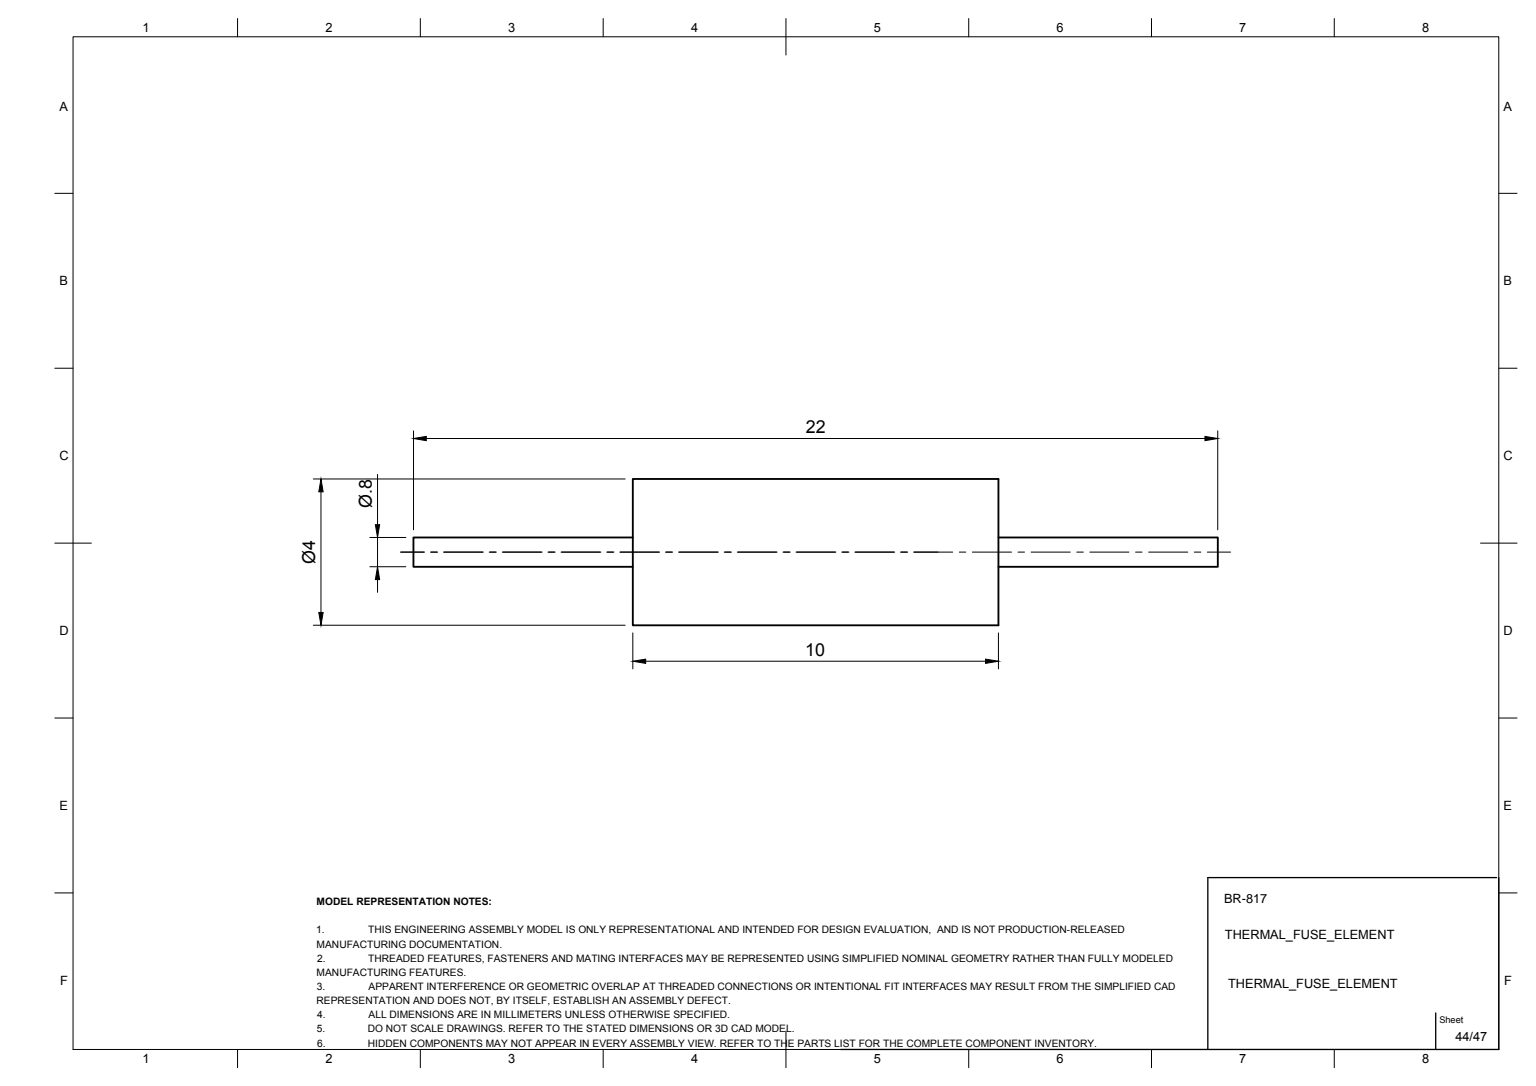
ISO-10303-21;
HEADER;
FILE_DESCRIPTION((''),'2;1');
FILE_NAME('THERMAL_FUSE_ELEMENT.step','2026-10-01T22:07:29-07:00',(''),(''),'','','');
FILE_SCHEMA (('AUTOMOTIVE_DESIGN { 1 0 10303 214 3 1 1 }'));
ENDSEC;
DATA;
#10=MECHANICAL_DESIGN_GEOMETRIC_PRESENTATION_REPRESENTATION('',(#579,#580,#581),#15484);
#504=SHAPE_REPRESENTATION_RELATIONSHIP('SRR','None',#15655,#539) ;
#539=ADVANCED_BREP_SHAPE_REPRESENTATION('',(#620,#621,#622),#15479) ;
#579=STYLED_ITEM('',(#15835),#620) ;
#580=STYLED_ITEM('',(#15842),#621) ;
#581=STYLED_ITEM('',(#15842),#622) ;
#620=MANIFOLD_SOLID_BREP('FUSE_BODY',#8290) ;
#621=MANIFOLD_SOLID_BREP('FUSE_LEADS',#8291) ;
#622=MANIFOLD_SOLID_BREP('FUSE_LEADS',#8292) ;
#802=CYLINDRICAL_SURFACE('',#9864,0.2) ;
#803=CYLINDRICAL_SURFACE('',#9869,0.04) ;
#804=CYLINDRICAL_SURFACE('',#9874,0.04) ;
#1349=CIRCLE('',#9865,0.2) ;
#1350=CIRCLE('',#9866,0.2) ;
#1351=CIRCLE('',#9870,0.04) ;
#1352=CIRCLE('',#9871,0.04) ;
#1353=CIRCLE('',#9875,0.04) ;
#1354=CIRCLE('',#9876,0.04) ;
#1843=FACE_OUTER_BOUND('',#2416,.T.) ;
#1844=FACE_OUTER_BOUND('',#2417,.T.) ;
#1845=FACE_OUTER_BOUND('',#2418,.T.) ;
#1846=FACE_OUTER_BOUND('',#2419,.T.) ;
#1847=FACE_OUTER_BOUND('',#2420,.T.) ;
#1848=FACE_OUTER_BOUND('',#2421,.T.) ;
#1849=FACE_OUTER_BOUND('',#2422,.T.) ;
#1850=FACE_OUTER_BOUND('',#2423,.T.) ;
#1851=FACE_OUTER_BOUND('',#2424,.T.) ;
#2416=EDGE_LOOP('',(#7489,#7490,#7491,#7492)) ;
#2417=EDGE_LOOP('',(#7493)) ;
#2418=EDGE_LOOP('',(#7494)) ;
#2419=EDGE_LOOP('',(#7495,#7496,#7497,#7498)) ;
#2420=EDGE_LOOP('',(#7499)) ;
#2421=EDGE_LOOP('',(#7500)) ;
#2422=EDGE_LOOP('',(#7501,#7502,#7503,#7504)) ;
#2423=EDGE_LOOP('',(#7505)) ;
#2424=EDGE_LOOP('',(#7506)) ;
#2906=LINE('',#15318,#3380) ;
#2907=LINE('',#15326,#3381) ;
#2908=LINE('',#15334,#3382) ;
#3380=VECTOR('',#12759,0.2) ;
#3381=VECTOR('',#12770,0.04) ;
#3382=VECTOR('',#12781,0.04) ;
#4125=VERTEX_POINT('',#15315) ;
#4126=VERTEX_POINT('',#15317) ;
#4127=VERTEX_POINT('',#15323) ;
#4128=VERTEX_POINT('',#15325) ;
#4129=VERTEX_POINT('',#15331) ;
#4130=VERTEX_POINT('',#15333) ;
#5249=EDGE_CURVE('',#4125,#4125,#1349,.T.) ;
#5250=EDGE_CURVE('',#4125,#4126,#2906,.T.) ;
#5251=EDGE_CURVE('',#4126,#4126,#1350,.T.) ;
#5252=EDGE_CURVE('',#4127,#4127,#1351,.T.) ;
#5253=EDGE_CURVE('',#4127,#4128,#2907,.T.) ;
#5254=EDGE_CURVE('',#4128,#4128,#1352,.T.) ;
#5255=EDGE_CURVE('',#4129,#4129,#1353,.T.) ;
#5256=EDGE_CURVE('',#4129,#4130,#2908,.T.) ;
#5257=EDGE_CURVE('',#4130,#4130,#1354,.T.) ;
#7489=ORIENTED_EDGE('',*,*,#5249,.F.) ;
#7490=ORIENTED_EDGE('',*,*,#5250,.T.) ;
#7491=ORIENTED_EDGE('',*,*,#5251,.F.) ;
#7492=ORIENTED_EDGE('',*,*,#5250,.F.) ;
#7493=ORIENTED_EDGE('',*,*,#5251,.T.) ;
#7494=ORIENTED_EDGE('',*,*,#5249,.T.) ;
#7495=ORIENTED_EDGE('',*,*,#5252,.F.) ;
#7496=ORIENTED_EDGE('',*,*,#5253,.T.) ;
#7497=ORIENTED_EDGE('',*,*,#5254,.F.) ;
#7498=ORIENTED_EDGE('',*,*,#5253,.F.) ;
#7499=ORIENTED_EDGE('',*,*,#5254,.T.) ;
#7500=ORIENTED_EDGE('',*,*,#5252,.T.) ;
#7501=ORIENTED_EDGE('',*,*,#5255,.F.) ;
#7502=ORIENTED_EDGE('',*,*,#5256,.T.) ;
#7503=ORIENTED_EDGE('',*,*,#5257,.F.) ;
#7504=ORIENTED_EDGE('',*,*,#5256,.F.) ;
#7505=ORIENTED_EDGE('',*,*,#5257,.T.) ;
#7506=ORIENTED_EDGE('',*,*,#5255,.T.) ;
#7738=PLANE('',#9867) ;
#7739=PLANE('',#9868) ;
#7740=PLANE('',#9872) ;
#7741=PLANE('',#9873) ;
#7742=PLANE('',#9877) ;
#7743=PLANE('',#9878) ;
#8230=ADVANCED_FACE('',(#1843),#802,.T.) ;
#8231=ADVANCED_FACE('',(#1844),#7738,.T.) ;
#8232=ADVANCED_FACE('',(#1845),#7739,.T.) ;
#8233=ADVANCED_FACE('',(#1846),#803,.T.) ;
#8234=ADVANCED_FACE('',(#1847),#7740,.T.) ;
#8235=ADVANCED_FACE('',(#1848),#7741,.T.) ;
#8236=ADVANCED_FACE('',(#1849),#804,.T.) ;
#8237=ADVANCED_FACE('',(#1850),#7742,.T.) ;
#8238=ADVANCED_FACE('',(#1851),#7743,.T.) ;
#8290=CLOSED_SHELL('',(#8230,#8231,#8232)) ;
#8291=CLOSED_SHELL('',(#8233,#8234,#8235)) ;
#8292=CLOSED_SHELL('',(#8236,#8237,#8238)) ;
#9863=AXIS2_PLACEMENT_3D('',#15313,#12753,#12754) ;
#9864=AXIS2_PLACEMENT_3D('',#15314,#12755,#12756) ;
#9865=AXIS2_PLACEMENT_3D('',#15316,#12757,#12758) ;
#9866=AXIS2_PLACEMENT_3D('',#15319,#12760,#12761) ;
#9867=AXIS2_PLACEMENT_3D('',#15320,#12762,#12763) ;
#9868=AXIS2_PLACEMENT_3D('',#15321,#12764,#12765) ;
#9869=AXIS2_PLACEMENT_3D('',#15322,#12766,#12767) ;
#9870=AXIS2_PLACEMENT_3D('',#15324,#12768,#12769) ;
#9871=AXIS2_PLACEMENT_3D('',#15327,#12771,#12772) ;
#9872=AXIS2_PLACEMENT_3D('',#15328,#12773,#12774) ;
#9873=AXIS2_PLACEMENT_3D('',#15329,#12775,#12776) ;
#9874=AXIS2_PLACEMENT_3D('',#15330,#12777,#12778) ;
#9875=AXIS2_PLACEMENT_3D('',#15332,#12779,#12780) ;
#9876=AXIS2_PLACEMENT_3D('',#15335,#12782,#12783) ;
#9877=AXIS2_PLACEMENT_3D('',#15336,#12784,#12785) ;
#9878=AXIS2_PLACEMENT_3D('',#15337,#12786,#12787) ;
#12753=DIRECTION('axis',(0.,0.,1.)) ;
#12754=DIRECTION('refdir',(1.,0.,0.)) ;
#12755=DIRECTION('center_axis',(1.,0.,0.)) ;
#12756=DIRECTION('ref_axis',(0.,0.,-1.)) ;
#12757=DIRECTION('center_axis',(1.,0.,0.)) ;
#12758=DIRECTION('ref_axis',(0.,0.,-1.)) ;
#12759=DIRECTION('',(-1.,0.,0.)) ;
#12760=DIRECTION('center_axis',(-1.,0.,0.)) ;
#12761=DIRECTION('ref_axis',(0.,0.,-1.)) ;
#12762=DIRECTION('center_axis',(-1.,0.,0.)) ;
#12763=DIRECTION('ref_axis',(0.,0.,1.)) ;
#12764=DIRECTION('center_axis',(1.,0.,0.)) ;
#12765=DIRECTION('ref_axis',(0.,0.,-1.)) ;
#12766=DIRECTION('center_axis',(1.,0.,0.)) ;
#12767=DIRECTION('ref_axis',(0.,0.,-1.)) ;
#12768=DIRECTION('center_axis',(1.,0.,0.)) ;
#12769=DIRECTION('ref_axis',(0.,0.,-1.)) ;
#12770=DIRECTION('',(-1.,0.,0.)) ;
#12771=DIRECTION('center_axis',(-1.,0.,0.)) ;
#12772=DIRECTION('ref_axis',(0.,0.,-1.)) ;
#12773=DIRECTION('center_axis',(-1.,0.,0.)) ;
#12774=DIRECTION('ref_axis',(0.,0.,1.)) ;
#12775=DIRECTION('center_axis',(1.,0.,0.)) ;
#12776=DIRECTION('ref_axis',(0.,0.,-1.)) ;
#12777=DIRECTION('center_axis',(1.,0.,0.)) ;
#12778=DIRECTION('ref_axis',(0.,0.,-1.)) ;
#12779=DIRECTION('center_axis',(1.,0.,0.)) ;
#12780=DIRECTION('ref_axis',(0.,0.,-1.)) ;
#12781=DIRECTION('',(-1.,0.,0.)) ;
#12782=DIRECTION('center_axis',(-1.,0.,0.)) ;
#12783=DIRECTION('ref_axis',(0.,0.,-1.)) ;
#12784=DIRECTION('center_axis',(-1.,0.,0.)) ;
#12785=DIRECTION('ref_axis',(0.,0.,1.)) ;
#12786=DIRECTION('center_axis',(1.,0.,0.)) ;
#12787=DIRECTION('ref_axis',(0.,0.,-1.)) ;
#15313=CARTESIAN_POINT('',(0.,0.,0.)) ;
#15314=CARTESIAN_POINT('Origin',(1.6,-1.8,0.6)) ;
#15315=CARTESIAN_POINT('',(2.1,-1.8,0.8)) ;
#15316=CARTESIAN_POINT('Origin',(2.1,-1.8,0.6)) ;
#15317=CARTESIAN_POINT('',(1.1,-1.8,0.8)) ;
#15318=CARTESIAN_POINT('',(1.6,-1.8,0.8)) ;
#15319=CARTESIAN_POINT('Origin',(1.1,-1.8,0.6)) ;
#15320=CARTESIAN_POINT('Origin',(1.1,-1.8,0.6)) ;
#15321=CARTESIAN_POINT('Origin',(2.1,-1.8,0.6)) ;
#15322=CARTESIAN_POINT('Origin',(0.8,-1.8,0.6)) ;
#15323=CARTESIAN_POINT('',(1.1,-1.8,0.64)) ;
#15324=CARTESIAN_POINT('Origin',(1.1,-1.8,0.6)) ;
#15325=CARTESIAN_POINT('',(0.5,-1.8,0.64)) ;
#15326=CARTESIAN_POINT('',(0.8,-1.8,0.64)) ;
#15327=CARTESIAN_POINT('Origin',(0.5,-1.8,0.6)) ;
#15328=CARTESIAN_POINT('Origin',(0.5,-1.8,0.6)) ;
#15329=CARTESIAN_POINT('Origin',(1.1,-1.8,0.6)) ;
#15330=CARTESIAN_POINT('Origin',(2.4,-1.8,0.6)) ;
#15331=CARTESIAN_POINT('',(2.7,-1.8,0.64)) ;
#15332=CARTESIAN_POINT('Origin',(2.7,-1.8,0.6)) ;
#15333=CARTESIAN_POINT('',(2.1,-1.8,0.64)) ;
#15334=CARTESIAN_POINT('',(2.4,-1.8,0.64)) ;
#15335=CARTESIAN_POINT('Origin',(2.1,-1.8,0.6)) ;
#15336=CARTESIAN_POINT('Origin',(2.1,-1.8,0.6)) ;
#15337=CARTESIAN_POINT('Origin',(2.7,-1.8,0.6)) ;
#15436=UNCERTAINTY_MEASURE_WITH_UNIT(LENGTH_MEASURE(0.001),#15485,
'DISTANCE_ACCURACY_VALUE',
'Maximum model space distance between geometric entities at asserted c
onnectivities') ;
#15441=UNCERTAINTY_MEASURE_WITH_UNIT(LENGTH_MEASURE(0.001),#15485,
'DISTANCE_ACCURACY_VALUE',
'Maximum model space distance between geometric entities at asserted c
onnectivities') ;
#15479=(
GEOMETRIC_REPRESENTATION_CONTEXT(3)
GLOBAL_UNCERTAINTY_ASSIGNED_CONTEXT((#15436))
GLOBAL_UNIT_ASSIGNED_CONTEXT((#15485,#15487,#15488))
REPRESENTATION_CONTEXT('','3D')
) ;
#15484=(
GEOMETRIC_REPRESENTATION_CONTEXT(3)
GLOBAL_UNCERTAINTY_ASSIGNED_CONTEXT((#15441))
GLOBAL_UNIT_ASSIGNED_CONTEXT((#15485,#15487,#15488))
REPRESENTATION_CONTEXT('','3D')
) ;
#15485=(
LENGTH_UNIT()
NAMED_UNIT(*)
SI_UNIT(.CENTI.,.METRE.)
) ;
#15487=(
NAMED_UNIT(*)
PLANE_ANGLE_UNIT()
SI_UNIT($,.RADIAN.)
) ;
#15488=(
NAMED_UNIT(*)
SI_UNIT($,.STERADIAN.)
SOLID_ANGLE_UNIT()
) ;
#15526=SHAPE_DEFINITION_REPRESENTATION(#15594,#15655) ;
#15594=PRODUCT_DEFINITION_SHAPE('',$,#15698) ;
#15655=SHAPE_REPRESENTATION('',(#9863),#15479) ;
#15660=PRODUCT_DEFINITION_CONTEXT('part definition',#15788,'design') ;
#15698=PRODUCT_DEFINITION('THERMAL_FUSE_ELEMENT',
'THERMAL_FUSE_ELEMENT',#15740,#15660) ;
#15740=PRODUCT_DEFINITION_FORMATION('',$,#15827) ;
#15788=APPLICATION_CONTEXT(
'Core Data for Automotive Mechanical Design Process') ;
#15789=PRODUCT_CONTEXT('part definition',#15788,'mechanical') ;
#15827=PRODUCT('THERMAL_FUSE_ELEMENT','THERMAL_FUSE_ELEMENT',$,(#15789)) ;
#15835=PRESENTATION_STYLE_ASSIGNMENT((#15847)) ;
#15842=PRESENTATION_STYLE_ASSIGNMENT((#15854)) ;
#15847=SURFACE_STYLE_USAGE(.BOTH.,#15859) ;
#15854=SURFACE_STYLE_USAGE(.BOTH.,#15866) ;
#15859=SURFACE_SIDE_STYLE('',(#15871)) ;
#15866=SURFACE_SIDE_STYLE('',(#15878)) ;
#15871=SURFACE_STYLE_FILL_AREA(#15883) ;
#15878=SURFACE_STYLE_FILL_AREA(#15890) ;
#15883=FILL_AREA_STYLE('Stainless Steel - Satin',(#15895)) ;
#15890=FILL_AREA_STYLE('Copper - Polished',(#15902)) ;
#15895=FILL_AREA_STYLE_COLOUR('Stainless Steel - Satin',#15907) ;
#15902=FILL_AREA_STYLE_COLOUR('Copper - Polished',#15914) ;
#15907=COLOUR_RGB('Stainless Steel - Satin', 0.40784314, 0.44705882, 0.49803922) ;
#15914=COLOUR_RGB('Copper - Polished', 0.66274510, 0.83137255, 0.94901961) ;
ENDSEC;
END-ISO-10303-21;
